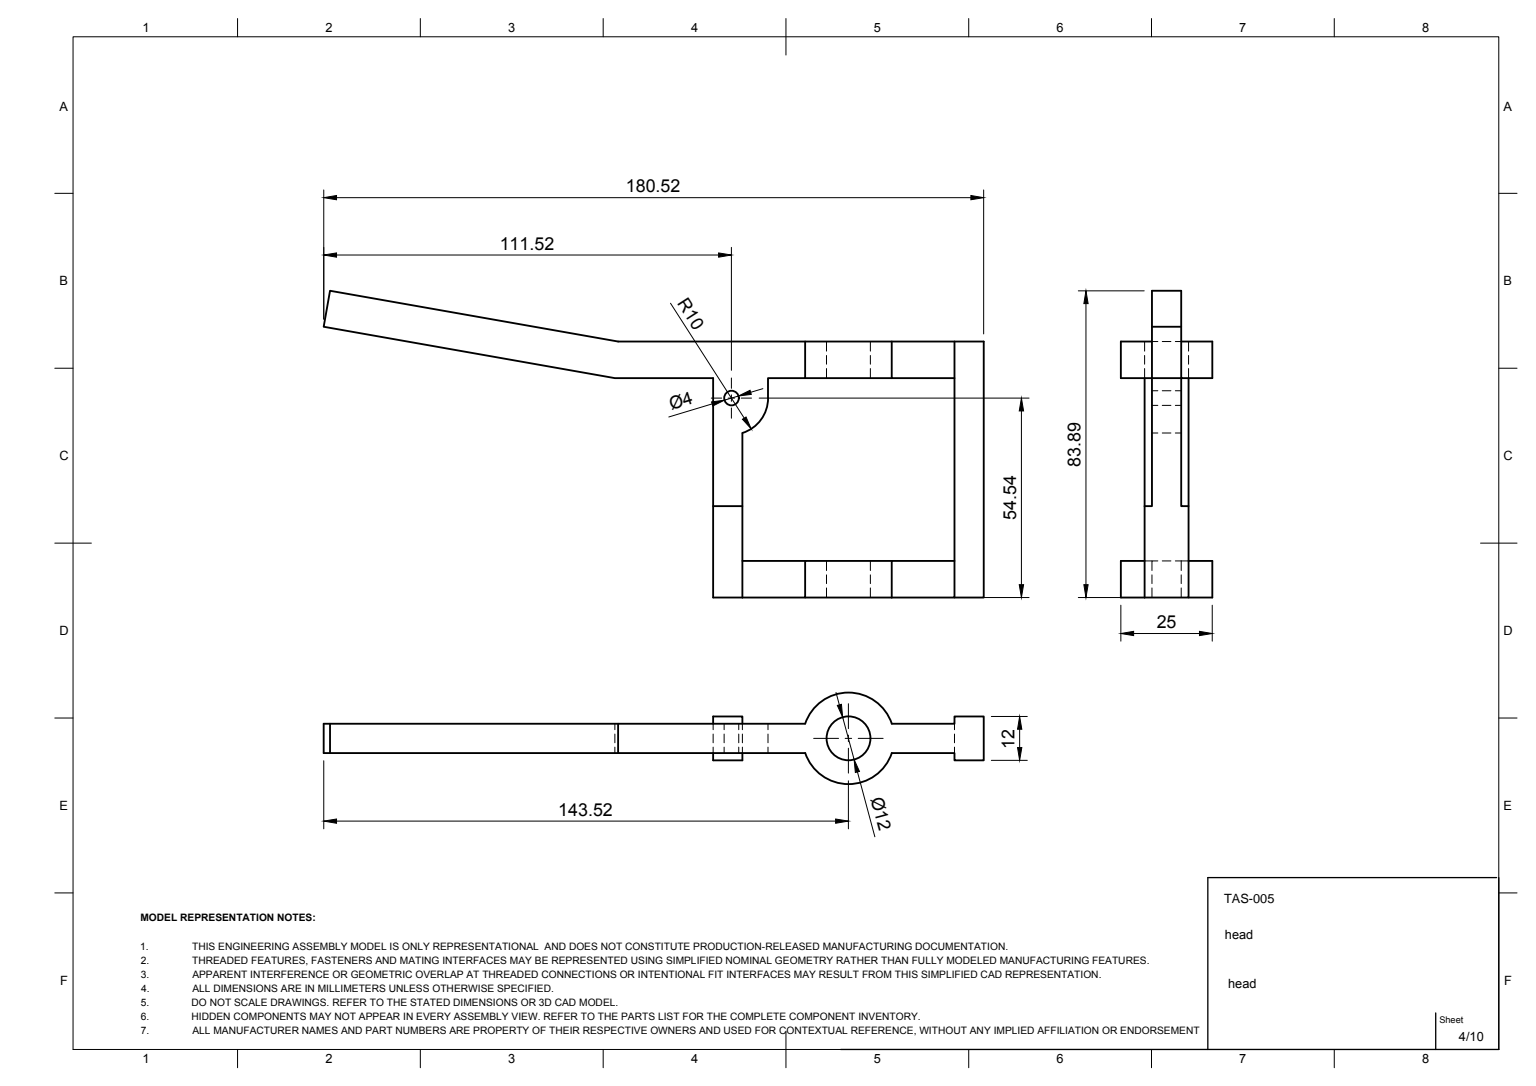
ISO-10303-21;
HEADER;
/* Generated by software containing ST-Developer
 * from STEP Tools, Inc. (www.steptools.com) 
 */

FILE_DESCRIPTION(
/* description */ ('STEP AP214'),
/* implementation_level */ '2;1');

FILE_NAME(
/* name */ 'head.step',
/* time_stamp */ '2026-11-04T19:54:22-08:00',
/* author */ (''),
/* organization */ (''),
/* preprocessor_version */ 'ST-DEVELOPER v20.2',
/* originating_system */ 'Autodesk Translation Framework v15.17.0.0',
/* authorisation */ '');

FILE_SCHEMA (('AUTOMOTIVE_DESIGN { 1 0 10303 214 3 1 1 }'));
ENDSEC;

DATA;
#10=MECHANICAL_DESIGN_GEOMETRIC_PRESENTATION_REPRESENTATION('',(#240),#14084);
#222=SHAPE_REPRESENTATION_RELATIONSHIP('SRR','None',#14121,#231);
#231=ADVANCED_BREP_SHAPE_REPRESENTATION('',(#249),#14076);
#240=STYLED_ITEM('',(#14175),#249);
#249=MANIFOLD_SOLID_BREP('Body1',#3466);
#259=FACE_BOUND('',#580,.T.);
#260=FACE_BOUND('',#590,.T.);
#261=FACE_BOUND('',#593,.T.);
#262=FACE_BOUND('',#599,.T.);
#263=FACE_BOUND('',#601,.T.);
#264=FACE_BOUND('',#603,.T.);
#297=PLANE('',#3613);
#298=PLANE('',#3614);
#299=PLANE('',#3615);
#300=PLANE('',#3617);
#301=PLANE('',#3618);
#302=PLANE('',#3619);
#303=PLANE('',#3620);
#304=PLANE('',#3621);
#305=PLANE('',#3622);
#306=PLANE('',#3623);
#307=PLANE('',#3624);
#308=PLANE('',#3625);
#309=PLANE('',#3627);
#310=PLANE('',#3628);
#311=PLANE('',#3631);
#312=PLANE('',#3632);
#313=PLANE('',#3633);
#314=PLANE('',#3634);
#315=PLANE('',#3636);
#316=PLANE('',#3638);
#317=PLANE('',#3640);
#318=PLANE('',#3641);
#319=PLANE('',#3642);
#320=PLANE('',#3643);
#321=PLANE('',#3645);
#322=PLANE('',#3646);
#323=PLANE('',#3647);
#380=FACE_OUTER_BOUND('',#572,.T.);
#381=FACE_OUTER_BOUND('',#573,.T.);
#382=FACE_OUTER_BOUND('',#574,.T.);
#383=FACE_OUTER_BOUND('',#575,.T.);
#384=FACE_OUTER_BOUND('',#576,.T.);
#385=FACE_OUTER_BOUND('',#577,.T.);
#386=FACE_OUTER_BOUND('',#578,.T.);
#387=FACE_OUTER_BOUND('',#579,.T.);
#388=FACE_OUTER_BOUND('',#581,.T.);
#389=FACE_OUTER_BOUND('',#582,.T.);
#390=FACE_OUTER_BOUND('',#583,.T.);
#391=FACE_OUTER_BOUND('',#584,.T.);
#392=FACE_OUTER_BOUND('',#585,.T.);
#393=FACE_OUTER_BOUND('',#586,.T.);
#394=FACE_OUTER_BOUND('',#587,.T.);
#395=FACE_OUTER_BOUND('',#588,.T.);
#396=FACE_OUTER_BOUND('',#589,.T.);
#397=FACE_OUTER_BOUND('',#591,.T.);
#398=FACE_OUTER_BOUND('',#592,.T.);
#399=FACE_OUTER_BOUND('',#594,.T.);
#400=FACE_OUTER_BOUND('',#595,.T.);
#401=FACE_OUTER_BOUND('',#596,.T.);
#402=FACE_OUTER_BOUND('',#597,.T.);
#403=FACE_OUTER_BOUND('',#598,.T.);
#404=FACE_OUTER_BOUND('',#600,.T.);
#405=FACE_OUTER_BOUND('',#602,.T.);
#406=FACE_OUTER_BOUND('',#604,.T.);
#407=FACE_OUTER_BOUND('',#605,.T.);
#408=FACE_OUTER_BOUND('',#606,.T.);
#409=FACE_OUTER_BOUND('',#607,.T.);
#410=FACE_OUTER_BOUND('',#608,.T.);
#411=FACE_OUTER_BOUND('',#609,.T.);
#412=FACE_OUTER_BOUND('',#610,.T.);
#413=FACE_OUTER_BOUND('',#611,.T.);
#414=FACE_OUTER_BOUND('',#612,.T.);
#572=EDGE_LOOP('',(#2275,#2276,#2277,#2278));
#573=EDGE_LOOP('',(#2279,#2280,#2281,#2282));
#574=EDGE_LOOP('',(#2283,#2284,#2285,#2286));
#575=EDGE_LOOP('',(#2287,#2288,#2289,#2290));
#576=EDGE_LOOP('',(#2291,#2292,#2293,#2294));
#577=EDGE_LOOP('',(#2295,#2296,#2297,#2298,#2299,#2300,#2301,#2302,#2303,
#2304,#2305,#2306));
#578=EDGE_LOOP('',(#2307,#2308,#2309,#2310));
#579=EDGE_LOOP('',(#2311,#2312,#2313,#2314,#2315,#2316,#2317,#2318,#2319,
#2320,#2321,#2322));
#580=EDGE_LOOP('',(#2323));
#581=EDGE_LOOP('',(#2324,#2325,#2326,#2327));
#582=EDGE_LOOP('',(#2328,#2329,#2330,#2331));
#583=EDGE_LOOP('',(#2332,#2333,#2334,#2335,#2336,#2337,#2338,#2339));
#584=EDGE_LOOP('',(#2340,#2341,#2342,#2343,#2344,#2345,#2346,#2347,#2348,
#2349,#2350,#2351));
#585=EDGE_LOOP('',(#2352,#2353,#2354,#2355));
#586=EDGE_LOOP('',(#2356,#2357,#2358,#2359));
#587=EDGE_LOOP('',(#2360,#2361,#2362,#2363));
#588=EDGE_LOOP('',(#2364,#2365,#2366,#2367));
#589=EDGE_LOOP('',(#2368,#2369,#2370,#2371,#2372,#2373,#2374,#2375));
#590=EDGE_LOOP('',(#2376));
#591=EDGE_LOOP('',(#2377,#2378,#2379,#2380));
#592=EDGE_LOOP('',(#2381,#2382,#2383,#2384,#2385,#2386,#2387,#2388,#2389,
#2390,#2391,#2392,#2393,#2394,#2395,#2396));
#593=EDGE_LOOP('',(#2397));
#594=EDGE_LOOP('',(#2398,#2399,#2400,#2401));
#595=EDGE_LOOP('',(#2402,#2403,#2404,#2405));
#596=EDGE_LOOP('',(#2406,#2407,#2408,#2409));
#597=EDGE_LOOP('',(#2410,#2411,#2412,#2413));
#598=EDGE_LOOP('',(#2414,#2415,#2416,#2417,#2418,#2419,#2420,#2421,#2422,
#2423,#2424,#2425));
#599=EDGE_LOOP('',(#2426));
#600=EDGE_LOOP('',(#2427,#2428,#2429,#2430,#2431,#2432,#2433,#2434,#2435,
#2436,#2437,#2438));
#601=EDGE_LOOP('',(#2439));
#602=EDGE_LOOP('',(#2440,#2441,#2442,#2443,#2444,#2445,#2446,#2447));
#603=EDGE_LOOP('',(#2448));
#604=EDGE_LOOP('',(#2449,#2450,#2451,#2452));
#605=EDGE_LOOP('',(#2453,#2454,#2455,#2456));
#606=EDGE_LOOP('',(#2457,#2458,#2459,#2460));
#607=EDGE_LOOP('',(#2461,#2462,#2463,#2464));
#608=EDGE_LOOP('',(#2465,#2466,#2467,#2468));
#609=EDGE_LOOP('',(#2469,#2470,#2471,#2472));
#610=EDGE_LOOP('',(#2473,#2474,#2475,#2476));
#611=EDGE_LOOP('',(#2477,#2478,#2479,#2480));
#612=EDGE_LOOP('',(#2481,#2482,#2483,#2484));
#806=LINE('',#4788,#1063);
#807=LINE('',#4794,#1064);
#808=LINE('',#4800,#1065);
#809=LINE('',#4807,#1066);
#810=LINE('',#4810,#1067);
#811=LINE('',#4816,#1068);
#812=LINE('',#4819,#1069);
#813=LINE('',#4823,#1070);
#814=LINE('',#4825,#1071);
#815=LINE('',#4827,#1072);
#816=LINE('',#4829,#1073);
#817=LINE('',#4831,#1074);
#818=LINE('',#4833,#1075);
#819=LINE('',#4835,#1076);
#820=LINE('',#4837,#1077);
#821=LINE('',#4839,#1078);
#822=LINE('',#4841,#1079);
#823=LINE('',#4843,#1080);
#824=LINE('',#4844,#1081);
#825=LINE('',#4847,#1082);
#826=LINE('',#4849,#1083);
#827=LINE('',#4850,#1084);
#828=LINE('',#4853,#1085);
#829=LINE('',#4855,#1086);
#830=LINE('',#4857,#1087);
#831=LINE('',#4861,#1088);
#832=LINE('',#4863,#1089);
#833=LINE('',#4865,#1090);
#834=LINE('',#4867,#1091);
#835=LINE('',#4869,#1092);
#836=LINE('',#4871,#1093);
#837=LINE('',#4872,#1094);
#838=LINE('',#4875,#1095);
#839=LINE('',#4876,#1096);
#840=LINE('',#4879,#1097);
#841=LINE('',#4881,#1098);
#842=LINE('',#4882,#1099);
#843=LINE('',#4886,#1100);
#844=LINE('',#4888,#1101);
#845=LINE('',#4889,#1102);
#846=LINE('',#4891,#1103);
#847=LINE('',#4893,#1104);
#848=LINE('',#4895,#1105);
#849=LINE('',#4896,#1106);
#850=LINE('',#4899,#1107);
#851=LINE('',#4901,#1108);
#852=LINE('',#4903,#1109);
#853=LINE('',#4905,#1110);
#854=LINE('',#4907,#1111);
#855=LINE('',#4909,#1112);
#856=LINE('',#4910,#1113);
#857=LINE('',#4911,#1114);
#858=LINE('',#4913,#1115);
#859=LINE('',#4914,#1116);
#860=LINE('',#4917,#1117);
#861=LINE('',#4919,#1118);
#862=LINE('',#4920,#1119);
#863=LINE('',#4922,#1120);
#864=LINE('',#4923,#1121);
#865=LINE('',#4926,#1122);
#866=LINE('',#4928,#1123);
#867=LINE('',#4929,#1124);
#868=LINE('',#4934,#1125);
#869=LINE('',#4936,#1126);
#870=LINE('',#4937,#1127);
#871=LINE('',#4939,#1128);
#872=LINE('',#4940,#1129);
#873=LINE('',#4942,#1130);
#874=LINE('',#4945,#1131);
#875=LINE('',#4951,#1132);
#876=LINE('',#4953,#1133);
#877=LINE('',#4955,#1134);
#878=LINE('',#4957,#1135);
#879=LINE('',#4959,#1136);
#880=LINE('',#4960,#1137);
#881=LINE('',#4961,#1138);
#882=LINE('',#4966,#1139);
#883=LINE('',#4968,#1140);
#884=LINE('',#4969,#1141);
#885=LINE('',#4971,#1142);
#886=LINE('',#4973,#1143);
#887=LINE('',#4975,#1144);
#888=LINE('',#4976,#1145);
#889=LINE('',#4977,#1146);
#890=LINE('',#4979,#1147);
#891=LINE('',#4982,#1148);
#892=LINE('',#4984,#1149);
#893=LINE('',#4986,#1150);
#894=LINE('',#4992,#1151);
#1063=VECTOR('',#3949,2.);
#1064=VECTOR('',#3956,6.);
#1065=VECTOR('',#3963,6.);
#1066=VECTOR('',#3970,1000.);
#1067=VECTOR('',#3973,1000.);
#1068=VECTOR('',#3978,1000.);
#1069=VECTOR('',#3981,1000.);
#1070=VECTOR('',#3984,1000.);
#1071=VECTOR('',#3985,1000.);
#1072=VECTOR('',#3986,1000.);
#1073=VECTOR('',#3987,1000.);
#1074=VECTOR('',#3988,1000.);
#1075=VECTOR('',#3989,1000.);
#1076=VECTOR('',#3990,1000.);
#1077=VECTOR('',#3991,1000.);
#1078=VECTOR('',#3992,1000.);
#1079=VECTOR('',#3993,1000.);
#1080=VECTOR('',#3994,1000.);
#1081=VECTOR('',#3995,1000.);
#1082=VECTOR('',#3998,1000.);
#1083=VECTOR('',#3999,1000.);
#1084=VECTOR('',#4000,1000.);
#1085=VECTOR('',#4003,1000.);
#1086=VECTOR('',#4004,1000.);
#1087=VECTOR('',#4005,1000.);
#1088=VECTOR('',#4008,1000.);
#1089=VECTOR('',#4009,1000.);
#1090=VECTOR('',#4010,1000.);
#1091=VECTOR('',#4011,1000.);
#1092=VECTOR('',#4012,1000.);
#1093=VECTOR('',#4013,1000.);
#1094=VECTOR('',#4014,1000.);
#1095=VECTOR('',#4017,1000.);
#1096=VECTOR('',#4018,1000.);
#1097=VECTOR('',#4021,1000.);
#1098=VECTOR('',#4022,1000.);
#1099=VECTOR('',#4023,1000.);
#1100=VECTOR('',#4026,1000.);
#1101=VECTOR('',#4027,1000.);
#1102=VECTOR('',#4028,1000.);
#1103=VECTOR('',#4029,1000.);
#1104=VECTOR('',#4030,1000.);
#1105=VECTOR('',#4031,1000.);
#1106=VECTOR('',#4032,1000.);
#1107=VECTOR('',#4035,1000.);
#1108=VECTOR('',#4036,1000.);
#1109=VECTOR('',#4037,1000.);
#1110=VECTOR('',#4038,1000.);
#1111=VECTOR('',#4039,1000.);
#1112=VECTOR('',#4040,1000.);
#1113=VECTOR('',#4041,1000.);
#1114=VECTOR('',#4042,1000.);
#1115=VECTOR('',#4045,1000.);
#1116=VECTOR('',#4046,1000.);
#1117=VECTOR('',#4049,1000.);
#1118=VECTOR('',#4050,1000.);
#1119=VECTOR('',#4051,1000.);
#1120=VECTOR('',#4054,1000.);
#1121=VECTOR('',#4055,1000.);
#1122=VECTOR('',#4058,1000.);
#1123=VECTOR('',#4059,1000.);
#1124=VECTOR('',#4060,1000.);
#1125=VECTOR('',#4067,1000.);
#1126=VECTOR('',#4068,1000.);
#1127=VECTOR('',#4069,1000.);
#1128=VECTOR('',#4072,1000.);
#1129=VECTOR('',#4073,1000.);
#1130=VECTOR('',#4076,1000.);
#1131=VECTOR('',#4081,1000.);
#1132=VECTOR('',#4088,1000.);
#1133=VECTOR('',#4091,1000.);
#1134=VECTOR('',#4092,1000.);
#1135=VECTOR('',#4093,1000.);
#1136=VECTOR('',#4094,1000.);
#1137=VECTOR('',#4095,1000.);
#1138=VECTOR('',#4096,1000.);
#1139=VECTOR('',#4101,1000.);
#1140=VECTOR('',#4102,1000.);
#1141=VECTOR('',#4103,1000.);
#1142=VECTOR('',#4104,1000.);
#1143=VECTOR('',#4105,1000.);
#1144=VECTOR('',#4106,1000.);
#1145=VECTOR('',#4107,1000.);
#1146=VECTOR('',#4108,1000.);
#1147=VECTOR('',#4111,1000.);
#1148=VECTOR('',#4116,1000.);
#1149=VECTOR('',#4119,1000.);
#1150=VECTOR('',#4122,1000.);
#1151=VECTOR('',#4133,1000.);
#1293=CIRCLE('',#3599,2.);
#1294=CIRCLE('',#3600,2.);
#1295=CIRCLE('',#3602,6.);
#1296=CIRCLE('',#3603,6.);
#1297=CIRCLE('',#3605,6.);
#1298=CIRCLE('',#3606,6.);
#1299=CIRCLE('',#3608,12.5);
#1300=CIRCLE('',#3609,12.5);
#1301=CIRCLE('',#3611,12.5);
#1302=CIRCLE('',#3612,12.5);
#1303=CIRCLE('',#3616,12.5);
#1304=CIRCLE('',#3626,12.5);
#1305=CIRCLE('',#3629,12.5);
#1306=CIRCLE('',#3635,10.);
#1307=CIRCLE('',#3637,10.);
#1308=CIRCLE('',#3639,12.5);
#1403=VERTEX_POINT('',#4785);
#1404=VERTEX_POINT('',#4787);
#1405=VERTEX_POINT('',#4791);
#1406=VERTEX_POINT('',#4793);
#1407=VERTEX_POINT('',#4797);
#1408=VERTEX_POINT('',#4799);
#1409=VERTEX_POINT('',#4803);
#1410=VERTEX_POINT('',#4804);
#1411=VERTEX_POINT('',#4806);
#1412=VERTEX_POINT('',#4808);
#1413=VERTEX_POINT('',#4812);
#1414=VERTEX_POINT('',#4813);
#1415=VERTEX_POINT('',#4815);
#1416=VERTEX_POINT('',#4817);
#1417=VERTEX_POINT('',#4821);
#1418=VERTEX_POINT('',#4822);
#1419=VERTEX_POINT('',#4824);
#1420=VERTEX_POINT('',#4826);
#1421=VERTEX_POINT('',#4828);
#1422=VERTEX_POINT('',#4830);
#1423=VERTEX_POINT('',#4832);
#1424=VERTEX_POINT('',#4834);
#1425=VERTEX_POINT('',#4836);
#1426=VERTEX_POINT('',#4838);
#1427=VERTEX_POINT('',#4840);
#1428=VERTEX_POINT('',#4842);
#1429=VERTEX_POINT('',#4846);
#1430=VERTEX_POINT('',#4848);
#1431=VERTEX_POINT('',#4852);
#1432=VERTEX_POINT('',#4854);
#1433=VERTEX_POINT('',#4856);
#1434=VERTEX_POINT('',#4858);
#1435=VERTEX_POINT('',#4860);
#1436=VERTEX_POINT('',#4862);
#1437=VERTEX_POINT('',#4864);
#1438=VERTEX_POINT('',#4866);
#1439=VERTEX_POINT('',#4868);
#1440=VERTEX_POINT('',#4870);
#1441=VERTEX_POINT('',#4874);
#1442=VERTEX_POINT('',#4878);
#1443=VERTEX_POINT('',#4880);
#1444=VERTEX_POINT('',#4884);
#1445=VERTEX_POINT('',#4885);
#1446=VERTEX_POINT('',#4887);
#1447=VERTEX_POINT('',#4890);
#1448=VERTEX_POINT('',#4892);
#1449=VERTEX_POINT('',#4894);
#1450=VERTEX_POINT('',#4898);
#1451=VERTEX_POINT('',#4900);
#1452=VERTEX_POINT('',#4902);
#1453=VERTEX_POINT('',#4904);
#1454=VERTEX_POINT('',#4906);
#1455=VERTEX_POINT('',#4908);
#1456=VERTEX_POINT('',#4916);
#1457=VERTEX_POINT('',#4918);
#1458=VERTEX_POINT('',#4925);
#1459=VERTEX_POINT('',#4927);
#1460=VERTEX_POINT('',#4933);
#1461=VERTEX_POINT('',#4935);
#1462=VERTEX_POINT('',#4949);
#1463=VERTEX_POINT('',#4950);
#1464=VERTEX_POINT('',#4954);
#1465=VERTEX_POINT('',#4956);
#1466=VERTEX_POINT('',#4958);
#1467=VERTEX_POINT('',#4963);
#1468=VERTEX_POINT('',#4965);
#1469=VERTEX_POINT('',#4967);
#1470=VERTEX_POINT('',#4970);
#1471=VERTEX_POINT('',#4972);
#1472=VERTEX_POINT('',#4974);
#1741=EDGE_CURVE('',#1403,#1403,#1293,.T.);
#1742=EDGE_CURVE('',#1403,#1404,#806,.T.);
#1743=EDGE_CURVE('',#1404,#1404,#1294,.T.);
#1744=EDGE_CURVE('',#1405,#1405,#1295,.T.);
#1745=EDGE_CURVE('',#1405,#1406,#807,.T.);
#1746=EDGE_CURVE('',#1406,#1406,#1296,.T.);
#1747=EDGE_CURVE('',#1407,#1407,#1297,.T.);
#1748=EDGE_CURVE('',#1407,#1408,#808,.T.);
#1749=EDGE_CURVE('',#1408,#1408,#1298,.T.);
#1750=EDGE_CURVE('',#1409,#1410,#1299,.T.);
#1751=EDGE_CURVE('',#1411,#1410,#809,.T.);
#1752=EDGE_CURVE('',#1412,#1411,#1300,.T.);
#1753=EDGE_CURVE('',#1409,#1412,#810,.T.);
#1754=EDGE_CURVE('',#1413,#1414,#1301,.T.);
#1755=EDGE_CURVE('',#1415,#1414,#811,.T.);
#1756=EDGE_CURVE('',#1416,#1415,#1302,.T.);
#1757=EDGE_CURVE('',#1413,#1416,#812,.T.);
#1758=EDGE_CURVE('',#1417,#1418,#813,.T.);
#1759=EDGE_CURVE('',#1418,#1419,#814,.T.);
#1760=EDGE_CURVE('',#1420,#1419,#815,.T.);
#1761=EDGE_CURVE('',#1421,#1420,#816,.T.);
#1762=EDGE_CURVE('',#1421,#1422,#817,.T.);
#1763=EDGE_CURVE('',#1422,#1423,#818,.T.);
#1764=EDGE_CURVE('',#1424,#1423,#819,.T.);
#1765=EDGE_CURVE('',#1424,#1425,#820,.T.);
#1766=EDGE_CURVE('',#1425,#1426,#821,.T.);
#1767=EDGE_CURVE('',#1426,#1427,#822,.T.);
#1768=EDGE_CURVE('',#1428,#1427,#823,.T.);
#1769=EDGE_CURVE('',#1417,#1428,#824,.T.);
#1770=EDGE_CURVE('',#1428,#1429,#825,.T.);
#1771=EDGE_CURVE('',#1427,#1430,#826,.T.);
#1772=EDGE_CURVE('',#1429,#1430,#827,.T.);
#1773=EDGE_CURVE('',#1411,#1431,#828,.T.);
#1774=EDGE_CURVE('',#1431,#1432,#829,.T.);
#1775=EDGE_CURVE('',#1433,#1432,#830,.T.);
#1776=EDGE_CURVE('',#1433,#1434,#1303,.T.);
#1777=EDGE_CURVE('',#1435,#1434,#831,.T.);
#1778=EDGE_CURVE('',#1435,#1436,#832,.T.);
#1779=EDGE_CURVE('',#1436,#1437,#833,.T.);
#1780=EDGE_CURVE('',#1437,#1438,#834,.T.);
#1781=EDGE_CURVE('',#1438,#1439,#835,.T.);
#1782=EDGE_CURVE('',#1439,#1440,#836,.T.);
#1783=EDGE_CURVE('',#1440,#1412,#837,.T.);
#1784=EDGE_CURVE('',#1441,#1409,#838,.T.);
#1785=EDGE_CURVE('',#1440,#1441,#839,.T.);
#1786=EDGE_CURVE('',#1442,#1434,#840,.T.);
#1787=EDGE_CURVE('',#1443,#1442,#841,.T.);
#1788=EDGE_CURVE('',#1435,#1443,#842,.T.);
#1789=EDGE_CURVE('',#1444,#1445,#843,.T.);
#1790=EDGE_CURVE('',#1446,#1445,#844,.T.);
#1791=EDGE_CURVE('',#1429,#1446,#845,.T.);
#1792=EDGE_CURVE('',#1447,#1430,#846,.T.);
#1793=EDGE_CURVE('',#1448,#1447,#847,.T.);
#1794=EDGE_CURVE('',#1449,#1448,#848,.T.);
#1795=EDGE_CURVE('',#1444,#1449,#849,.T.);
#1796=EDGE_CURVE('',#1439,#1450,#850,.T.);
#1797=EDGE_CURVE('',#1450,#1451,#851,.T.);
#1798=EDGE_CURVE('',#1451,#1452,#852,.T.);
#1799=EDGE_CURVE('',#1452,#1453,#853,.T.);
#1800=EDGE_CURVE('',#1454,#1453,#854,.T.);
#1801=EDGE_CURVE('',#1454,#1455,#855,.T.);
#1802=EDGE_CURVE('',#1436,#1455,#856,.T.);
#1803=EDGE_CURVE('',#1441,#1443,#857,.T.);
#1804=EDGE_CURVE('',#1451,#1413,#858,.T.);
#1805=EDGE_CURVE('',#1452,#1416,#859,.T.);
#1806=EDGE_CURVE('',#1454,#1456,#860,.T.);
#1807=EDGE_CURVE('',#1453,#1457,#861,.T.);
#1808=EDGE_CURVE('',#1456,#1457,#862,.T.);
#1809=EDGE_CURVE('',#1415,#1425,#863,.T.);
#1810=EDGE_CURVE('',#1414,#1426,#864,.T.);
#1811=EDGE_CURVE('',#1458,#1424,#865,.T.);
#1812=EDGE_CURVE('',#1459,#1423,#866,.T.);
#1813=EDGE_CURVE('',#1458,#1459,#867,.T.);
#1814=EDGE_CURVE('',#1458,#1457,#1304,.T.);
#1815=EDGE_CURVE('',#1438,#1460,#868,.T.);
#1816=EDGE_CURVE('',#1437,#1461,#869,.T.);
#1817=EDGE_CURVE('',#1460,#1461,#870,.T.);
#1818=EDGE_CURVE('',#1460,#1450,#871,.T.);
#1819=EDGE_CURVE('',#1455,#1461,#872,.T.);
#1820=EDGE_CURVE('',#1459,#1456,#1305,.T.);
#1821=EDGE_CURVE('',#1447,#1422,#873,.T.);
#1822=EDGE_CURVE('',#1421,#1448,#874,.T.);
#1823=EDGE_CURVE('',#1462,#1463,#875,.T.);
#1824=EDGE_CURVE('',#1463,#1418,#1306,.T.);
#1825=EDGE_CURVE('',#1417,#1446,#876,.T.);
#1826=EDGE_CURVE('',#1445,#1464,#877,.T.);
#1827=EDGE_CURVE('',#1464,#1465,#878,.T.);
#1828=EDGE_CURVE('',#1466,#1465,#879,.T.);
#1829=EDGE_CURVE('',#1431,#1466,#880,.T.);
#1830=EDGE_CURVE('',#1410,#1462,#881,.T.);
#1831=EDGE_CURVE('',#1419,#1467,#1307,.T.);
#1832=EDGE_CURVE('',#1468,#1467,#882,.T.);
#1833=EDGE_CURVE('',#1469,#1468,#883,.T.);
#1834=EDGE_CURVE('',#1433,#1469,#884,.T.);
#1835=EDGE_CURVE('',#1432,#1470,#885,.T.);
#1836=EDGE_CURVE('',#1470,#1471,#886,.T.);
#1837=EDGE_CURVE('',#1472,#1471,#887,.T.);
#1838=EDGE_CURVE('',#1444,#1472,#888,.T.);
#1839=EDGE_CURVE('',#1420,#1449,#889,.T.);
#1840=EDGE_CURVE('',#1468,#1462,#890,.T.);
#1841=EDGE_CURVE('',#1469,#1442,#1308,.T.);
#1842=EDGE_CURVE('',#1464,#1472,#891,.T.);
#1843=EDGE_CURVE('',#1465,#1471,#892,.T.);
#1844=EDGE_CURVE('',#1466,#1470,#893,.T.);
#1845=EDGE_CURVE('',#1467,#1463,#894,.T.);
#2275=ORIENTED_EDGE('',*,*,#1741,.T.);
#2276=ORIENTED_EDGE('',*,*,#1742,.T.);
#2277=ORIENTED_EDGE('',*,*,#1743,.F.);
#2278=ORIENTED_EDGE('',*,*,#1742,.F.);
#2279=ORIENTED_EDGE('',*,*,#1744,.F.);
#2280=ORIENTED_EDGE('',*,*,#1745,.T.);
#2281=ORIENTED_EDGE('',*,*,#1746,.F.);
#2282=ORIENTED_EDGE('',*,*,#1745,.F.);
#2283=ORIENTED_EDGE('',*,*,#1747,.F.);
#2284=ORIENTED_EDGE('',*,*,#1748,.T.);
#2285=ORIENTED_EDGE('',*,*,#1749,.T.);
#2286=ORIENTED_EDGE('',*,*,#1748,.F.);
#2287=ORIENTED_EDGE('',*,*,#1750,.T.);
#2288=ORIENTED_EDGE('',*,*,#1751,.F.);
#2289=ORIENTED_EDGE('',*,*,#1752,.F.);
#2290=ORIENTED_EDGE('',*,*,#1753,.F.);
#2291=ORIENTED_EDGE('',*,*,#1754,.T.);
#2292=ORIENTED_EDGE('',*,*,#1755,.F.);
#2293=ORIENTED_EDGE('',*,*,#1756,.F.);
#2294=ORIENTED_EDGE('',*,*,#1757,.F.);
#2295=ORIENTED_EDGE('',*,*,#1758,.T.);
#2296=ORIENTED_EDGE('',*,*,#1759,.T.);
#2297=ORIENTED_EDGE('',*,*,#1760,.F.);
#2298=ORIENTED_EDGE('',*,*,#1761,.F.);
#2299=ORIENTED_EDGE('',*,*,#1762,.T.);
#2300=ORIENTED_EDGE('',*,*,#1763,.T.);
#2301=ORIENTED_EDGE('',*,*,#1764,.F.);
#2302=ORIENTED_EDGE('',*,*,#1765,.T.);
#2303=ORIENTED_EDGE('',*,*,#1766,.T.);
#2304=ORIENTED_EDGE('',*,*,#1767,.T.);
#2305=ORIENTED_EDGE('',*,*,#1768,.F.);
#2306=ORIENTED_EDGE('',*,*,#1769,.F.);
#2307=ORIENTED_EDGE('',*,*,#1770,.F.);
#2308=ORIENTED_EDGE('',*,*,#1768,.T.);
#2309=ORIENTED_EDGE('',*,*,#1771,.T.);
#2310=ORIENTED_EDGE('',*,*,#1772,.F.);
#2311=ORIENTED_EDGE('',*,*,#1752,.T.);
#2312=ORIENTED_EDGE('',*,*,#1773,.T.);
#2313=ORIENTED_EDGE('',*,*,#1774,.T.);
#2314=ORIENTED_EDGE('',*,*,#1775,.F.);
#2315=ORIENTED_EDGE('',*,*,#1776,.T.);
#2316=ORIENTED_EDGE('',*,*,#1777,.F.);
#2317=ORIENTED_EDGE('',*,*,#1778,.T.);
#2318=ORIENTED_EDGE('',*,*,#1779,.T.);
#2319=ORIENTED_EDGE('',*,*,#1780,.T.);
#2320=ORIENTED_EDGE('',*,*,#1781,.T.);
#2321=ORIENTED_EDGE('',*,*,#1782,.T.);
#2322=ORIENTED_EDGE('',*,*,#1783,.T.);
#2323=ORIENTED_EDGE('',*,*,#1749,.F.);
#2324=ORIENTED_EDGE('',*,*,#1784,.T.);
#2325=ORIENTED_EDGE('',*,*,#1753,.T.);
#2326=ORIENTED_EDGE('',*,*,#1783,.F.);
#2327=ORIENTED_EDGE('',*,*,#1785,.T.);
#2328=ORIENTED_EDGE('',*,*,#1786,.F.);
#2329=ORIENTED_EDGE('',*,*,#1787,.F.);
#2330=ORIENTED_EDGE('',*,*,#1788,.F.);
#2331=ORIENTED_EDGE('',*,*,#1777,.T.);
#2332=ORIENTED_EDGE('',*,*,#1789,.T.);
#2333=ORIENTED_EDGE('',*,*,#1790,.F.);
#2334=ORIENTED_EDGE('',*,*,#1791,.F.);
#2335=ORIENTED_EDGE('',*,*,#1772,.T.);
#2336=ORIENTED_EDGE('',*,*,#1792,.F.);
#2337=ORIENTED_EDGE('',*,*,#1793,.F.);
#2338=ORIENTED_EDGE('',*,*,#1794,.F.);
#2339=ORIENTED_EDGE('',*,*,#1795,.F.);
#2340=ORIENTED_EDGE('',*,*,#1785,.F.);
#2341=ORIENTED_EDGE('',*,*,#1782,.F.);
#2342=ORIENTED_EDGE('',*,*,#1796,.T.);
#2343=ORIENTED_EDGE('',*,*,#1797,.T.);
#2344=ORIENTED_EDGE('',*,*,#1798,.T.);
#2345=ORIENTED_EDGE('',*,*,#1799,.T.);
#2346=ORIENTED_EDGE('',*,*,#1800,.F.);
#2347=ORIENTED_EDGE('',*,*,#1801,.T.);
#2348=ORIENTED_EDGE('',*,*,#1802,.F.);
#2349=ORIENTED_EDGE('',*,*,#1778,.F.);
#2350=ORIENTED_EDGE('',*,*,#1788,.T.);
#2351=ORIENTED_EDGE('',*,*,#1803,.F.);
#2352=ORIENTED_EDGE('',*,*,#1798,.F.);
#2353=ORIENTED_EDGE('',*,*,#1804,.T.);
#2354=ORIENTED_EDGE('',*,*,#1757,.T.);
#2355=ORIENTED_EDGE('',*,*,#1805,.F.);
#2356=ORIENTED_EDGE('',*,*,#1806,.F.);
#2357=ORIENTED_EDGE('',*,*,#1800,.T.);
#2358=ORIENTED_EDGE('',*,*,#1807,.T.);
#2359=ORIENTED_EDGE('',*,*,#1808,.F.);
#2360=ORIENTED_EDGE('',*,*,#1766,.F.);
#2361=ORIENTED_EDGE('',*,*,#1809,.F.);
#2362=ORIENTED_EDGE('',*,*,#1755,.T.);
#2363=ORIENTED_EDGE('',*,*,#1810,.T.);
#2364=ORIENTED_EDGE('',*,*,#1811,.T.);
#2365=ORIENTED_EDGE('',*,*,#1764,.T.);
#2366=ORIENTED_EDGE('',*,*,#1812,.F.);
#2367=ORIENTED_EDGE('',*,*,#1813,.F.);
#2368=ORIENTED_EDGE('',*,*,#1799,.F.);
#2369=ORIENTED_EDGE('',*,*,#1805,.T.);
#2370=ORIENTED_EDGE('',*,*,#1756,.T.);
#2371=ORIENTED_EDGE('',*,*,#1809,.T.);
#2372=ORIENTED_EDGE('',*,*,#1765,.F.);
#2373=ORIENTED_EDGE('',*,*,#1811,.F.);
#2374=ORIENTED_EDGE('',*,*,#1814,.T.);
#2375=ORIENTED_EDGE('',*,*,#1807,.F.);
#2376=ORIENTED_EDGE('',*,*,#1746,.T.);
#2377=ORIENTED_EDGE('',*,*,#1815,.F.);
#2378=ORIENTED_EDGE('',*,*,#1780,.F.);
#2379=ORIENTED_EDGE('',*,*,#1816,.T.);
#2380=ORIENTED_EDGE('',*,*,#1817,.F.);
#2381=ORIENTED_EDGE('',*,*,#1792,.T.);
#2382=ORIENTED_EDGE('',*,*,#1771,.F.);
#2383=ORIENTED_EDGE('',*,*,#1767,.F.);
#2384=ORIENTED_EDGE('',*,*,#1810,.F.);
#2385=ORIENTED_EDGE('',*,*,#1754,.F.);
#2386=ORIENTED_EDGE('',*,*,#1804,.F.);
#2387=ORIENTED_EDGE('',*,*,#1797,.F.);
#2388=ORIENTED_EDGE('',*,*,#1818,.F.);
#2389=ORIENTED_EDGE('',*,*,#1817,.T.);
#2390=ORIENTED_EDGE('',*,*,#1819,.F.);
#2391=ORIENTED_EDGE('',*,*,#1801,.F.);
#2392=ORIENTED_EDGE('',*,*,#1806,.T.);
#2393=ORIENTED_EDGE('',*,*,#1820,.F.);
#2394=ORIENTED_EDGE('',*,*,#1812,.T.);
#2395=ORIENTED_EDGE('',*,*,#1763,.F.);
#2396=ORIENTED_EDGE('',*,*,#1821,.F.);
#2397=ORIENTED_EDGE('',*,*,#1744,.T.);
#2398=ORIENTED_EDGE('',*,*,#1820,.T.);
#2399=ORIENTED_EDGE('',*,*,#1808,.T.);
#2400=ORIENTED_EDGE('',*,*,#1814,.F.);
#2401=ORIENTED_EDGE('',*,*,#1813,.T.);
#2402=ORIENTED_EDGE('',*,*,#1762,.F.);
#2403=ORIENTED_EDGE('',*,*,#1822,.T.);
#2404=ORIENTED_EDGE('',*,*,#1793,.T.);
#2405=ORIENTED_EDGE('',*,*,#1821,.T.);
#2406=ORIENTED_EDGE('',*,*,#1818,.T.);
#2407=ORIENTED_EDGE('',*,*,#1796,.F.);
#2408=ORIENTED_EDGE('',*,*,#1781,.F.);
#2409=ORIENTED_EDGE('',*,*,#1815,.T.);
#2410=ORIENTED_EDGE('',*,*,#1819,.T.);
#2411=ORIENTED_EDGE('',*,*,#1816,.F.);
#2412=ORIENTED_EDGE('',*,*,#1779,.F.);
#2413=ORIENTED_EDGE('',*,*,#1802,.T.);
#2414=ORIENTED_EDGE('',*,*,#1823,.T.);
#2415=ORIENTED_EDGE('',*,*,#1824,.T.);
#2416=ORIENTED_EDGE('',*,*,#1758,.F.);
#2417=ORIENTED_EDGE('',*,*,#1825,.T.);
#2418=ORIENTED_EDGE('',*,*,#1790,.T.);
#2419=ORIENTED_EDGE('',*,*,#1826,.T.);
#2420=ORIENTED_EDGE('',*,*,#1827,.T.);
#2421=ORIENTED_EDGE('',*,*,#1828,.F.);
#2422=ORIENTED_EDGE('',*,*,#1829,.F.);
#2423=ORIENTED_EDGE('',*,*,#1773,.F.);
#2424=ORIENTED_EDGE('',*,*,#1751,.T.);
#2425=ORIENTED_EDGE('',*,*,#1830,.T.);
#2426=ORIENTED_EDGE('',*,*,#1743,.T.);
#2427=ORIENTED_EDGE('',*,*,#1760,.T.);
#2428=ORIENTED_EDGE('',*,*,#1831,.T.);
#2429=ORIENTED_EDGE('',*,*,#1832,.F.);
#2430=ORIENTED_EDGE('',*,*,#1833,.F.);
#2431=ORIENTED_EDGE('',*,*,#1834,.F.);
#2432=ORIENTED_EDGE('',*,*,#1775,.T.);
#2433=ORIENTED_EDGE('',*,*,#1835,.T.);
#2434=ORIENTED_EDGE('',*,*,#1836,.T.);
#2435=ORIENTED_EDGE('',*,*,#1837,.F.);
#2436=ORIENTED_EDGE('',*,*,#1838,.F.);
#2437=ORIENTED_EDGE('',*,*,#1795,.T.);
#2438=ORIENTED_EDGE('',*,*,#1839,.F.);
#2439=ORIENTED_EDGE('',*,*,#1741,.F.);
#2440=ORIENTED_EDGE('',*,*,#1833,.T.);
#2441=ORIENTED_EDGE('',*,*,#1840,.T.);
#2442=ORIENTED_EDGE('',*,*,#1830,.F.);
#2443=ORIENTED_EDGE('',*,*,#1750,.F.);
#2444=ORIENTED_EDGE('',*,*,#1784,.F.);
#2445=ORIENTED_EDGE('',*,*,#1803,.T.);
#2446=ORIENTED_EDGE('',*,*,#1787,.T.);
#2447=ORIENTED_EDGE('',*,*,#1841,.F.);
#2448=ORIENTED_EDGE('',*,*,#1747,.T.);
#2449=ORIENTED_EDGE('',*,*,#1789,.F.);
#2450=ORIENTED_EDGE('',*,*,#1838,.T.);
#2451=ORIENTED_EDGE('',*,*,#1842,.F.);
#2452=ORIENTED_EDGE('',*,*,#1826,.F.);
#2453=ORIENTED_EDGE('',*,*,#1837,.T.);
#2454=ORIENTED_EDGE('',*,*,#1843,.F.);
#2455=ORIENTED_EDGE('',*,*,#1827,.F.);
#2456=ORIENTED_EDGE('',*,*,#1842,.T.);
#2457=ORIENTED_EDGE('',*,*,#1836,.F.);
#2458=ORIENTED_EDGE('',*,*,#1844,.F.);
#2459=ORIENTED_EDGE('',*,*,#1828,.T.);
#2460=ORIENTED_EDGE('',*,*,#1843,.T.);
#2461=ORIENTED_EDGE('',*,*,#1835,.F.);
#2462=ORIENTED_EDGE('',*,*,#1774,.F.);
#2463=ORIENTED_EDGE('',*,*,#1829,.T.);
#2464=ORIENTED_EDGE('',*,*,#1844,.T.);
#2465=ORIENTED_EDGE('',*,*,#1841,.T.);
#2466=ORIENTED_EDGE('',*,*,#1786,.T.);
#2467=ORIENTED_EDGE('',*,*,#1776,.F.);
#2468=ORIENTED_EDGE('',*,*,#1834,.T.);
#2469=ORIENTED_EDGE('',*,*,#1761,.T.);
#2470=ORIENTED_EDGE('',*,*,#1839,.T.);
#2471=ORIENTED_EDGE('',*,*,#1794,.T.);
#2472=ORIENTED_EDGE('',*,*,#1822,.F.);
#2473=ORIENTED_EDGE('',*,*,#1769,.T.);
#2474=ORIENTED_EDGE('',*,*,#1770,.T.);
#2475=ORIENTED_EDGE('',*,*,#1791,.T.);
#2476=ORIENTED_EDGE('',*,*,#1825,.F.);
#2477=ORIENTED_EDGE('',*,*,#1832,.T.);
#2478=ORIENTED_EDGE('',*,*,#1845,.T.);
#2479=ORIENTED_EDGE('',*,*,#1823,.F.);
#2480=ORIENTED_EDGE('',*,*,#1840,.F.);
#2481=ORIENTED_EDGE('',*,*,#1831,.F.);
#2482=ORIENTED_EDGE('',*,*,#1759,.F.);
#2483=ORIENTED_EDGE('',*,*,#1824,.F.);
#2484=ORIENTED_EDGE('',*,*,#1845,.F.);
#3190=CYLINDRICAL_SURFACE('',#3598,2.);
#3191=CYLINDRICAL_SURFACE('',#3601,6.);
#3192=CYLINDRICAL_SURFACE('',#3604,6.);
#3193=CYLINDRICAL_SURFACE('',#3607,12.5);
#3194=CYLINDRICAL_SURFACE('',#3610,12.5);
#3195=CYLINDRICAL_SURFACE('',#3630,12.5);
#3196=CYLINDRICAL_SURFACE('',#3644,12.5);
#3197=CYLINDRICAL_SURFACE('',#3648,10.);
#3290=ADVANCED_FACE('',(#380),#3190,.F.);
#3291=ADVANCED_FACE('',(#381),#3191,.F.);
#3292=ADVANCED_FACE('',(#382),#3192,.F.);
#3293=ADVANCED_FACE('',(#383),#3193,.T.);
#3294=ADVANCED_FACE('',(#384),#3194,.T.);
#3295=ADVANCED_FACE('',(#385),#297,.F.);
#3296=ADVANCED_FACE('',(#386),#298,.F.);
#3297=ADVANCED_FACE('',(#387,#259),#299,.T.);
#3298=ADVANCED_FACE('',(#388),#300,.F.);
#3299=ADVANCED_FACE('',(#389),#301,.T.);
#3300=ADVANCED_FACE('',(#390),#302,.T.);
#3301=ADVANCED_FACE('',(#391),#303,.F.);
#3302=ADVANCED_FACE('',(#392),#304,.F.);
#3303=ADVANCED_FACE('',(#393),#305,.T.);
#3304=ADVANCED_FACE('',(#394),#306,.F.);
#3305=ADVANCED_FACE('',(#395),#307,.T.);
#3306=ADVANCED_FACE('',(#396,#260),#308,.F.);
#3307=ADVANCED_FACE('',(#397),#309,.T.);
#3308=ADVANCED_FACE('',(#398,#261),#310,.T.);
#3309=ADVANCED_FACE('',(#399),#3195,.T.);
#3310=ADVANCED_FACE('',(#400),#311,.F.);
#3311=ADVANCED_FACE('',(#401),#312,.F.);
#3312=ADVANCED_FACE('',(#402),#313,.F.);
#3313=ADVANCED_FACE('',(#403,#262),#314,.F.);
#3314=ADVANCED_FACE('',(#404,#263),#315,.T.);
#3315=ADVANCED_FACE('',(#405,#264),#316,.F.);
#3316=ADVANCED_FACE('',(#406),#317,.F.);
#3317=ADVANCED_FACE('',(#407),#318,.F.);
#3318=ADVANCED_FACE('',(#408),#319,.T.);
#3319=ADVANCED_FACE('',(#409),#320,.T.);
#3320=ADVANCED_FACE('',(#410),#3196,.T.);
#3321=ADVANCED_FACE('',(#411),#321,.F.);
#3322=ADVANCED_FACE('',(#412),#322,.F.);
#3323=ADVANCED_FACE('',(#413),#323,.T.);
#3324=ADVANCED_FACE('',(#414),#3197,.T.);
#3466=CLOSED_SHELL('',(#3290,#3291,#3292,#3293,#3294,#3295,#3296,#3297,
#3298,#3299,#3300,#3301,#3302,#3303,#3304,#3305,#3306,#3307,#3308,#3309,
#3310,#3311,#3312,#3313,#3314,#3315,#3316,#3317,#3318,#3319,#3320,#3321,
#3322,#3323,#3324));
#3597=AXIS2_PLACEMENT_3D('',#4783,#3943,#3944);
#3598=AXIS2_PLACEMENT_3D('',#4784,#3945,#3946);
#3599=AXIS2_PLACEMENT_3D('',#4786,#3947,#3948);
#3600=AXIS2_PLACEMENT_3D('',#4789,#3950,#3951);
#3601=AXIS2_PLACEMENT_3D('',#4790,#3952,#3953);
#3602=AXIS2_PLACEMENT_3D('',#4792,#3954,#3955);
#3603=AXIS2_PLACEMENT_3D('',#4795,#3957,#3958);
#3604=AXIS2_PLACEMENT_3D('',#4796,#3959,#3960);
#3605=AXIS2_PLACEMENT_3D('',#4798,#3961,#3962);
#3606=AXIS2_PLACEMENT_3D('',#4801,#3964,#3965);
#3607=AXIS2_PLACEMENT_3D('',#4802,#3966,#3967);
#3608=AXIS2_PLACEMENT_3D('',#4805,#3968,#3969);
#3609=AXIS2_PLACEMENT_3D('',#4809,#3971,#3972);
#3610=AXIS2_PLACEMENT_3D('',#4811,#3974,#3975);
#3611=AXIS2_PLACEMENT_3D('',#4814,#3976,#3977);
#3612=AXIS2_PLACEMENT_3D('',#4818,#3979,#3980);
#3613=AXIS2_PLACEMENT_3D('',#4820,#3982,#3983);
#3614=AXIS2_PLACEMENT_3D('',#4845,#3996,#3997);
#3615=AXIS2_PLACEMENT_3D('',#4851,#4001,#4002);
#3616=AXIS2_PLACEMENT_3D('',#4859,#4006,#4007);
#3617=AXIS2_PLACEMENT_3D('',#4873,#4015,#4016);
#3618=AXIS2_PLACEMENT_3D('',#4877,#4019,#4020);
#3619=AXIS2_PLACEMENT_3D('',#4883,#4024,#4025);
#3620=AXIS2_PLACEMENT_3D('',#4897,#4033,#4034);
#3621=AXIS2_PLACEMENT_3D('',#4912,#4043,#4044);
#3622=AXIS2_PLACEMENT_3D('',#4915,#4047,#4048);
#3623=AXIS2_PLACEMENT_3D('',#4921,#4052,#4053);
#3624=AXIS2_PLACEMENT_3D('',#4924,#4056,#4057);
#3625=AXIS2_PLACEMENT_3D('',#4930,#4061,#4062);
#3626=AXIS2_PLACEMENT_3D('',#4931,#4063,#4064);
#3627=AXIS2_PLACEMENT_3D('',#4932,#4065,#4066);
#3628=AXIS2_PLACEMENT_3D('',#4938,#4070,#4071);
#3629=AXIS2_PLACEMENT_3D('',#4941,#4074,#4075);
#3630=AXIS2_PLACEMENT_3D('',#4943,#4077,#4078);
#3631=AXIS2_PLACEMENT_3D('',#4944,#4079,#4080);
#3632=AXIS2_PLACEMENT_3D('',#4946,#4082,#4083);
#3633=AXIS2_PLACEMENT_3D('',#4947,#4084,#4085);
#3634=AXIS2_PLACEMENT_3D('',#4948,#4086,#4087);
#3635=AXIS2_PLACEMENT_3D('',#4952,#4089,#4090);
#3636=AXIS2_PLACEMENT_3D('',#4962,#4097,#4098);
#3637=AXIS2_PLACEMENT_3D('',#4964,#4099,#4100);
#3638=AXIS2_PLACEMENT_3D('',#4978,#4109,#4110);
#3639=AXIS2_PLACEMENT_3D('',#4980,#4112,#4113);
#3640=AXIS2_PLACEMENT_3D('',#4981,#4114,#4115);
#3641=AXIS2_PLACEMENT_3D('',#4983,#4117,#4118);
#3642=AXIS2_PLACEMENT_3D('',#4985,#4120,#4121);
#3643=AXIS2_PLACEMENT_3D('',#4987,#4123,#4124);
#3644=AXIS2_PLACEMENT_3D('',#4988,#4125,#4126);
#3645=AXIS2_PLACEMENT_3D('',#4989,#4127,#4128);
#3646=AXIS2_PLACEMENT_3D('',#4990,#4129,#4130);
#3647=AXIS2_PLACEMENT_3D('',#4991,#4131,#4132);
#3648=AXIS2_PLACEMENT_3D('',#4993,#4134,#4135);
#3943=DIRECTION('axis',(0.,0.,1.));
#3944=DIRECTION('refdir',(1.,0.,0.));
#3945=DIRECTION('center_axis',(0.,0.,1.));
#3946=DIRECTION('ref_axis',(1.,0.,0.));
#3947=DIRECTION('center_axis',(0.,0.,-1.));
#3948=DIRECTION('ref_axis',(-1.,0.,0.));
#3949=DIRECTION('',(0.,0.,1.));
#3950=DIRECTION('center_axis',(0.,0.,-1.));
#3951=DIRECTION('ref_axis',(-1.,0.,0.));
#3952=DIRECTION('center_axis',(0.,1.,0.));
#3953=DIRECTION('ref_axis',(0.,0.,1.));
#3954=DIRECTION('center_axis',(0.,1.,0.));
#3955=DIRECTION('ref_axis',(0.,0.,1.));
#3956=DIRECTION('',(0.,1.,0.));
#3957=DIRECTION('center_axis',(0.,-1.,0.));
#3958=DIRECTION('ref_axis',(0.,0.,-1.));
#3959=DIRECTION('center_axis',(0.,1.,0.));
#3960=DIRECTION('ref_axis',(0.,0.,1.));
#3961=DIRECTION('center_axis',(0.,1.,0.));
#3962=DIRECTION('ref_axis',(0.,0.,1.));
#3963=DIRECTION('',(0.,1.,0.));
#3964=DIRECTION('center_axis',(0.,1.,0.));
#3965=DIRECTION('ref_axis',(0.,0.,1.));
#3966=DIRECTION('center_axis',(0.,1.,0.));
#3967=DIRECTION('ref_axis',(0.,0.,1.));
#3968=DIRECTION('center_axis',(0.,1.,0.));
#3969=DIRECTION('ref_axis',(0.,0.,1.));
#3970=DIRECTION('',(0.,-1.,0.));
#3971=DIRECTION('center_axis',(0.,1.,0.));
#3972=DIRECTION('ref_axis',(0.,0.,1.));
#3973=DIRECTION('',(0.,1.,0.));
#3974=DIRECTION('center_axis',(0.,1.,0.));
#3975=DIRECTION('ref_axis',(0.,0.,1.));
#3976=DIRECTION('center_axis',(0.,1.,0.));
#3977=DIRECTION('ref_axis',(0.,0.,1.));
#3978=DIRECTION('',(0.,-1.,0.));
#3979=DIRECTION('center_axis',(0.,1.,0.));
#3980=DIRECTION('ref_axis',(0.,0.,1.));
#3981=DIRECTION('',(0.,1.,0.));
#3982=DIRECTION('center_axis',(1.,0.,0.));
#3983=DIRECTION('ref_axis',(0.,0.,-1.));
#3984=DIRECTION('',(0.,1.,0.));
#3985=DIRECTION('',(0.,0.,-1.));
#3986=DIRECTION('',(0.,1.,0.));
#3987=DIRECTION('',(0.,0.,1.));
#3988=DIRECTION('',(0.,-1.,0.));
#3989=DIRECTION('',(0.,0.,1.));
#3990=DIRECTION('',(0.,-1.,0.));
#3991=DIRECTION('',(0.,0.,1.));
#3992=DIRECTION('',(0.,-1.,0.));
#3993=DIRECTION('',(0.,0.,1.));
#3994=DIRECTION('',(0.,-1.,0.));
#3995=DIRECTION('',(0.,0.,1.));
#3996=DIRECTION('center_axis',(-2.16840434497101E-16,0.,-1.));
#3997=DIRECTION('ref_axis',(-1.,0.,2.16840434497101E-16));
#3998=DIRECTION('',(1.,0.,0.));
#3999=DIRECTION('',(1.,0.,-2.16840434497101E-16));
#4000=DIRECTION('',(0.,-1.,0.));
#4001=DIRECTION('center_axis',(0.,1.,0.));
#4002=DIRECTION('ref_axis',(0.,0.,1.));
#4003=DIRECTION('',(1.,0.,0.));
#4004=DIRECTION('',(0.,0.,-1.));
#4005=DIRECTION('',(1.,0.,0.));
#4006=DIRECTION('center_axis',(0.,1.,0.));
#4007=DIRECTION('ref_axis',(0.,0.,1.));
#4008=DIRECTION('',(1.,0.,0.));
#4009=DIRECTION('',(0.,0.,-1.));
#4010=DIRECTION('',(-1.,0.,0.));
#4011=DIRECTION('',(0.,0.,1.));
#4012=DIRECTION('',(1.,0.,0.));
#4013=DIRECTION('',(0.,0.,-1.));
#4014=DIRECTION('',(1.,0.,0.));
#4015=DIRECTION('center_axis',(0.,0.,-1.));
#4016=DIRECTION('ref_axis',(-1.,0.,0.));
#4017=DIRECTION('',(1.,0.,0.));
#4018=DIRECTION('',(0.,-1.,0.));
#4019=DIRECTION('center_axis',(0.,0.,-1.));
#4020=DIRECTION('ref_axis',(-1.,0.,0.));
#4021=DIRECTION('',(0.,1.,0.));
#4022=DIRECTION('',(1.,0.,0.));
#4023=DIRECTION('',(0.,-1.,0.));
#4024=DIRECTION('center_axis',(1.,0.,0.));
#4025=DIRECTION('ref_axis',(0.,0.,-1.));
#4026=DIRECTION('',(0.,0.,1.));
#4027=DIRECTION('',(0.,1.,0.));
#4028=DIRECTION('',(0.,0.,-1.));
#4029=DIRECTION('',(0.,0.,1.));
#4030=DIRECTION('',(0.,-1.,0.));
#4031=DIRECTION('',(0.,0.,-1.));
#4032=DIRECTION('',(0.,-1.,0.));
#4033=DIRECTION('center_axis',(-1.,0.,0.));
#4034=DIRECTION('ref_axis',(0.,0.,1.));
#4035=DIRECTION('',(0.,-1.,0.));
#4036=DIRECTION('',(0.,0.,-1.));
#4037=DIRECTION('',(0.,1.,0.));
#4038=DIRECTION('',(0.,0.,-1.));
#4039=DIRECTION('',(0.,1.,0.));
#4040=DIRECTION('',(0.,0.,-1.));
#4041=DIRECTION('',(0.,-1.,0.));
#4042=DIRECTION('',(0.,0.,-1.));
#4043=DIRECTION('center_axis',(0.,0.,-1.));
#4044=DIRECTION('ref_axis',(-1.,0.,0.));
#4045=DIRECTION('',(1.,0.,0.));
#4046=DIRECTION('',(1.,0.,0.));
#4047=DIRECTION('center_axis',(0.,0.,-1.));
#4048=DIRECTION('ref_axis',(-1.,0.,0.));
#4049=DIRECTION('',(1.,0.,0.));
#4050=DIRECTION('',(1.,0.,0.));
#4051=DIRECTION('',(0.,1.,0.));
#4052=DIRECTION('center_axis',(0.,0.,-1.));
#4053=DIRECTION('ref_axis',(-1.,0.,0.));
#4054=DIRECTION('',(1.,0.,0.));
#4055=DIRECTION('',(1.,0.,0.));
#4056=DIRECTION('center_axis',(0.,0.,-1.));
#4057=DIRECTION('ref_axis',(-1.,0.,0.));
#4058=DIRECTION('',(1.,0.,0.));
#4059=DIRECTION('',(1.,0.,0.));
#4060=DIRECTION('',(0.,-1.,0.));
#4061=DIRECTION('center_axis',(0.,-1.,0.));
#4062=DIRECTION('ref_axis',(-1.,0.,0.));
#4063=DIRECTION('center_axis',(0.,1.,0.));
#4064=DIRECTION('ref_axis',(0.,0.,1.));
#4065=DIRECTION('center_axis',(-1.,0.,0.));
#4066=DIRECTION('ref_axis',(0.,0.,1.));
#4067=DIRECTION('',(0.,-1.,0.));
#4068=DIRECTION('',(0.,-1.,0.));
#4069=DIRECTION('',(0.,0.,-1.));
#4070=DIRECTION('center_axis',(0.,-1.,0.));
#4071=DIRECTION('ref_axis',(-1.,0.,0.));
#4072=DIRECTION('',(1.,0.,0.));
#4073=DIRECTION('',(-1.,0.,0.));
#4074=DIRECTION('center_axis',(0.,1.,0.));
#4075=DIRECTION('ref_axis',(0.,0.,1.));
#4076=DIRECTION('',(-1.,0.,2.16840434497101E-16));
#4077=DIRECTION('center_axis',(0.,1.,0.));
#4078=DIRECTION('ref_axis',(1.22464679914735E-16,0.,-1.));
#4079=DIRECTION('center_axis',(2.16840434497101E-16,0.,1.));
#4080=DIRECTION('ref_axis',(1.,0.,-2.16840434497101E-16));
#4081=DIRECTION('',(1.,0.,0.));
#4082=DIRECTION('center_axis',(0.,0.,-1.));
#4083=DIRECTION('ref_axis',(-1.,0.,0.));
#4084=DIRECTION('center_axis',(0.,0.,1.));
#4085=DIRECTION('ref_axis',(1.,0.,0.));
#4086=DIRECTION('center_axis',(0.,0.,-1.));
#4087=DIRECTION('ref_axis',(-1.,0.,0.));
#4088=DIRECTION('',(0.,-1.,0.));
#4089=DIRECTION('center_axis',(0.,0.,1.));
#4090=DIRECTION('ref_axis',(-1.,0.,0.));
#4091=DIRECTION('',(1.,0.,0.));
#4092=DIRECTION('',(1.,0.,0.));
#4093=DIRECTION('',(0.984807753012208,0.173648177666931,0.));
#4094=DIRECTION('',(0.173648177666933,-0.984807753012208,0.));
#4095=DIRECTION('',(0.984807753012208,0.173648177666931,0.));
#4096=DIRECTION('',(1.,0.,0.));
#4097=DIRECTION('center_axis',(0.,0.,-1.));
#4098=DIRECTION('ref_axis',(-1.,0.,0.));
#4099=DIRECTION('center_axis',(0.,0.,-1.));
#4100=DIRECTION('ref_axis',(-1.,0.,0.));
#4101=DIRECTION('',(0.,-1.,0.));
#4102=DIRECTION('',(1.,0.,0.));
#4103=DIRECTION('',(0.,-1.,0.));
#4104=DIRECTION('',(0.984807753012208,0.173648177666931,0.));
#4105=DIRECTION('',(0.173648177666933,-0.984807753012208,0.));
#4106=DIRECTION('',(0.984807753012208,0.173648177666931,0.));
#4107=DIRECTION('',(1.,0.,0.));
#4108=DIRECTION('',(1.,0.,0.));
#4109=DIRECTION('center_axis',(0.,1.,0.));
#4110=DIRECTION('ref_axis',(0.,0.,1.));
#4111=DIRECTION('',(0.,0.,1.));
#4112=DIRECTION('center_axis',(0.,1.,0.));
#4113=DIRECTION('ref_axis',(0.,0.,1.));
#4114=DIRECTION('center_axis',(0.,1.,0.));
#4115=DIRECTION('ref_axis',(0.,0.,1.));
#4116=DIRECTION('',(0.,0.,-1.));
#4117=DIRECTION('center_axis',(-0.173648177666931,0.984807753012208,0.));
#4118=DIRECTION('ref_axis',(-0.984807753012208,-0.173648177666931,0.));
#4119=DIRECTION('',(0.,0.,-1.));
#4120=DIRECTION('center_axis',(0.984807753012208,0.173648177666933,0.));
#4121=DIRECTION('ref_axis',(-0.173648177666933,0.984807753012208,0.));
#4122=DIRECTION('',(0.,0.,-1.));
#4123=DIRECTION('center_axis',(-0.173648177666931,0.984807753012208,0.));
#4124=DIRECTION('ref_axis',(-0.984807753012208,-0.173648177666931,0.));
#4125=DIRECTION('center_axis',(0.,1.,0.));
#4126=DIRECTION('ref_axis',(1.22464679914735E-16,0.,-1.));
#4127=DIRECTION('center_axis',(0.,-1.,0.));
#4128=DIRECTION('ref_axis',(0.,0.,-1.));
#4129=DIRECTION('center_axis',(0.,-1.,0.));
#4130=DIRECTION('ref_axis',(0.,0.,-1.));
#4131=DIRECTION('center_axis',(-1.,0.,0.));
#4132=DIRECTION('ref_axis',(0.,0.,1.));
#4133=DIRECTION('',(0.,0.,1.));
#4134=DIRECTION('center_axis',(0.,0.,1.));
#4135=DIRECTION('ref_axis',(1.,0.,0.));
#4783=CARTESIAN_POINT('',(0.,0.,0.));
#4784=CARTESIAN_POINT('Origin',(32.,329.539392014169,6.2));
#4785=CARTESIAN_POINT('',(30.,329.539392014169,-4.));
#4786=CARTESIAN_POINT('Origin',(32.,329.539392014169,-4.));
#4787=CARTESIAN_POINT('',(30.,329.539392014169,4.));
#4788=CARTESIAN_POINT('',(30.,329.539392014169,6.2));
#4789=CARTESIAN_POINT('Origin',(32.,329.539392014169,4.));
#4790=CARTESIAN_POINT('Origin',(0.,275.,0.));
#4791=CARTESIAN_POINT('',(-7.34788079488412E-16,275.,-6.));
#4792=CARTESIAN_POINT('Origin',(0.,275.,0.));
#4793=CARTESIAN_POINT('',(-7.34788079488412E-16,285.,-6.));
#4794=CARTESIAN_POINT('',(-7.34788079488412E-16,275.,-6.));
#4795=CARTESIAN_POINT('Origin',(0.,285.,0.));
#4796=CARTESIAN_POINT('Origin',(0.,275.,0.));
#4797=CARTESIAN_POINT('',(-7.34788079488412E-16,335.,-6.));
#4798=CARTESIAN_POINT('Origin',(0.,335.,0.));
#4799=CARTESIAN_POINT('',(-7.34788079488412E-16,345.,-6.));
#4800=CARTESIAN_POINT('',(-7.34788079488412E-16,275.,-6.));
#4801=CARTESIAN_POINT('Origin',(0.,345.,0.));
#4802=CARTESIAN_POINT('Origin',(0.,335.,0.));
#4803=CARTESIAN_POINT('',(-11.842719282327,335.,4.));
#4804=CARTESIAN_POINT('',(11.842719282327,335.,4.));
#4805=CARTESIAN_POINT('Origin',(0.,335.,0.));
#4806=CARTESIAN_POINT('',(11.842719282327,345.,4.));
#4807=CARTESIAN_POINT('',(11.842719282327,335.,4.));
#4808=CARTESIAN_POINT('',(-11.842719282327,345.,4.));
#4809=CARTESIAN_POINT('Origin',(0.,345.,0.));
#4810=CARTESIAN_POINT('',(-11.842719282327,335.,4.));
#4811=CARTESIAN_POINT('Origin',(0.,275.,0.));
#4812=CARTESIAN_POINT('',(-11.842719282327,275.,4.));
#4813=CARTESIAN_POINT('',(11.842719282327,275.,4.));
#4814=CARTESIAN_POINT('Origin',(0.,275.,0.));
#4815=CARTESIAN_POINT('',(11.842719282327,285.,4.));
#4816=CARTESIAN_POINT('',(11.842719282327,275.,4.));
#4817=CARTESIAN_POINT('',(-11.842719282327,285.,4.));
#4818=CARTESIAN_POINT('Origin',(0.,285.,0.));
#4819=CARTESIAN_POINT('',(-11.842719282327,275.,4.));
#4820=CARTESIAN_POINT('Origin',(29.,345.,-5.99999999999999));
#4821=CARTESIAN_POINT('',(29.,300.,4.));
#4822=CARTESIAN_POINT('',(29.,320.,4.));
#4823=CARTESIAN_POINT('',(29.,345.,4.));
#4824=CARTESIAN_POINT('',(29.,320.,-4.));
#4825=CARTESIAN_POINT('',(29.,320.,-5.99999999999999));
#4826=CARTESIAN_POINT('',(29.,300.,-4.));
#4827=CARTESIAN_POINT('',(29.,345.,-4.));
#4828=CARTESIAN_POINT('',(29.,300.,-6.));
#4829=CARTESIAN_POINT('',(29.,300.,-4.));
#4830=CARTESIAN_POINT('',(29.,275.,-5.99999999999999));
#4831=CARTESIAN_POINT('',(29.,345.,-5.99999999999999));
#4832=CARTESIAN_POINT('',(29.,275.,-4.));
#4833=CARTESIAN_POINT('',(29.,275.,-5.99999999999999));
#4834=CARTESIAN_POINT('',(29.,285.,-4.));
#4835=CARTESIAN_POINT('',(29.,285.,-4.));
#4836=CARTESIAN_POINT('',(29.,285.,4.));
#4837=CARTESIAN_POINT('',(29.,285.,0.));
#4838=CARTESIAN_POINT('',(29.,275.,4.));
#4839=CARTESIAN_POINT('',(29.,285.,4.));
#4840=CARTESIAN_POINT('',(29.,275.,6.00000000000001));
#4841=CARTESIAN_POINT('',(29.,275.,-5.99999999999999));
#4842=CARTESIAN_POINT('',(29.,300.,6.));
#4843=CARTESIAN_POINT('',(29.,345.,6.00000000000001));
#4844=CARTESIAN_POINT('',(29.,300.,4.));
#4845=CARTESIAN_POINT('Origin',(37.,345.,6.));
#4846=CARTESIAN_POINT('',(37.,300.,6.));
#4847=CARTESIAN_POINT('',(-37.001,300.,6.));
#4848=CARTESIAN_POINT('',(37.,275.,6.));
#4849=CARTESIAN_POINT('',(37.,275.,6.));
#4850=CARTESIAN_POINT('',(37.,345.,6.));
#4851=CARTESIAN_POINT('Origin',(0.,345.,0.));
#4852=CARTESIAN_POINT('',(63.,345.,4.));
#4853=CARTESIAN_POINT('',(-37.,345.,4.));
#4854=CARTESIAN_POINT('',(63.,345.,-4.));
#4855=CARTESIAN_POINT('',(63.,345.,4.));
#4856=CARTESIAN_POINT('',(11.842719282327,345.,-4.));
#4857=CARTESIAN_POINT('',(-37.,345.,-4.));
#4858=CARTESIAN_POINT('',(-11.842719282327,345.,-4.));
#4859=CARTESIAN_POINT('Origin',(0.,345.,0.));
#4860=CARTESIAN_POINT('',(-29.,345.,-4.));
#4861=CARTESIAN_POINT('',(-37.,345.,-4.));
#4862=CARTESIAN_POINT('',(-29.,345.,-5.99999999999999));
#4863=CARTESIAN_POINT('',(-29.,345.,-5.99999999999999));
#4864=CARTESIAN_POINT('',(-37.,345.,-5.99999999999999));
#4865=CARTESIAN_POINT('',(-37.,345.,-5.99999999999999));
#4866=CARTESIAN_POINT('',(-37.,345.,6.00000000000001));
#4867=CARTESIAN_POINT('',(-37.,345.,-5.99999999999999));
#4868=CARTESIAN_POINT('',(-29.,345.,6.00000000000001));
#4869=CARTESIAN_POINT('',(-37.,345.,6.00000000000001));
#4870=CARTESIAN_POINT('',(-29.,345.,4.));
#4871=CARTESIAN_POINT('',(-29.,345.,-5.99999999999999));
#4872=CARTESIAN_POINT('',(-37.,345.,4.));
#4873=CARTESIAN_POINT('Origin',(0.,0.,4.));
#4874=CARTESIAN_POINT('',(-29.,335.,4.));
#4875=CARTESIAN_POINT('',(-37.,335.,4.));
#4876=CARTESIAN_POINT('',(-29.,345.,4.));
#4877=CARTESIAN_POINT('Origin',(0.,0.,-4.));
#4878=CARTESIAN_POINT('',(-11.842719282327,335.,-4.));
#4879=CARTESIAN_POINT('',(-11.842719282327,335.,-4.));
#4880=CARTESIAN_POINT('',(-29.,335.,-4.));
#4881=CARTESIAN_POINT('',(-37.,335.,-4.));
#4882=CARTESIAN_POINT('',(-29.,345.,-4.));
#4883=CARTESIAN_POINT('Origin',(37.,285.,-4.));
#4884=CARTESIAN_POINT('',(37.,335.,-4.));
#4885=CARTESIAN_POINT('',(37.,335.,4.));
#4886=CARTESIAN_POINT('',(37.,335.,-4.));
#4887=CARTESIAN_POINT('',(37.,300.,4.));
#4888=CARTESIAN_POINT('',(37.,345.,4.));
#4889=CARTESIAN_POINT('',(37.,300.,4.));
#4890=CARTESIAN_POINT('',(37.,275.,-6.));
#4891=CARTESIAN_POINT('',(37.,275.,-4.));
#4892=CARTESIAN_POINT('',(37.,300.,-6.));
#4893=CARTESIAN_POINT('',(37.,345.,-6.));
#4894=CARTESIAN_POINT('',(37.,300.,-4.));
#4895=CARTESIAN_POINT('',(37.,300.,-4.));
#4896=CARTESIAN_POINT('',(37.,345.,-4.));
#4897=CARTESIAN_POINT('Origin',(-29.,345.,-5.99999999999999));
#4898=CARTESIAN_POINT('',(-29.,275.,6.00000000000001));
#4899=CARTESIAN_POINT('',(-29.,345.,6.00000000000001));
#4900=CARTESIAN_POINT('',(-29.,275.,4.));
#4901=CARTESIAN_POINT('',(-29.,275.,-5.99999999999999));
#4902=CARTESIAN_POINT('',(-29.,285.,4.));
#4903=CARTESIAN_POINT('',(-29.,285.,4.));
#4904=CARTESIAN_POINT('',(-29.,285.,-4.));
#4905=CARTESIAN_POINT('',(-29.,285.,0.));
#4906=CARTESIAN_POINT('',(-29.,275.,-4.));
#4907=CARTESIAN_POINT('',(-29.,285.,-4.));
#4908=CARTESIAN_POINT('',(-29.,275.,-5.99999999999999));
#4909=CARTESIAN_POINT('',(-29.,275.,-5.99999999999999));
#4910=CARTESIAN_POINT('',(-29.,345.,-5.99999999999999));
#4911=CARTESIAN_POINT('',(-29.,335.,-5.99999999999999));
#4912=CARTESIAN_POINT('Origin',(-37.,285.,4.));
#4913=CARTESIAN_POINT('',(-37.,275.,4.));
#4914=CARTESIAN_POINT('',(-37.,285.,4.));
#4915=CARTESIAN_POINT('Origin',(-37.,285.,-4.));
#4916=CARTESIAN_POINT('',(-11.842719282327,275.,-4.));
#4917=CARTESIAN_POINT('',(-37.,275.,-4.));
#4918=CARTESIAN_POINT('',(-11.842719282327,285.,-4.));
#4919=CARTESIAN_POINT('',(-37.,285.,-4.));
#4920=CARTESIAN_POINT('',(-11.842719282327,275.,-4.));
#4921=CARTESIAN_POINT('Origin',(-37.,285.,4.));
#4922=CARTESIAN_POINT('',(-37.,285.,4.));
#4923=CARTESIAN_POINT('',(-37.,275.,4.));
#4924=CARTESIAN_POINT('Origin',(-37.,285.,-4.));
#4925=CARTESIAN_POINT('',(11.842719282327,285.,-4.));
#4926=CARTESIAN_POINT('',(-37.,285.,-4.));
#4927=CARTESIAN_POINT('',(11.842719282327,275.,-4.));
#4928=CARTESIAN_POINT('',(-37.,275.,-4.));
#4929=CARTESIAN_POINT('',(11.842719282327,275.,-4.));
#4930=CARTESIAN_POINT('Origin',(0.,285.,0.));
#4931=CARTESIAN_POINT('Origin',(0.,285.,0.));
#4932=CARTESIAN_POINT('Origin',(-37.,285.,4.));
#4933=CARTESIAN_POINT('',(-37.,275.,6.00000000000001));
#4934=CARTESIAN_POINT('',(-37.,345.,6.00000000000001));
#4935=CARTESIAN_POINT('',(-37.,275.,-5.99999999999999));
#4936=CARTESIAN_POINT('',(-37.,345.,-5.99999999999999));
#4937=CARTESIAN_POINT('',(-37.,275.,4.));
#4938=CARTESIAN_POINT('Origin',(0.,275.,0.));
#4939=CARTESIAN_POINT('',(-37.,275.,6.00000000000001));
#4940=CARTESIAN_POINT('',(-37.,275.,-5.99999999999999));
#4941=CARTESIAN_POINT('Origin',(0.,275.,0.));
#4942=CARTESIAN_POINT('',(37.,275.,-6.));
#4943=CARTESIAN_POINT('Origin',(0.,275.,0.));
#4944=CARTESIAN_POINT('Origin',(37.,345.,-6.));
#4945=CARTESIAN_POINT('',(-37.001,300.,-6.));
#4946=CARTESIAN_POINT('Origin',(-37.,345.,6.00000000000001));
#4947=CARTESIAN_POINT('Origin',(-37.,345.,-5.99999999999999));
#4948=CARTESIAN_POINT('Origin',(0.,0.,4.));
#4949=CARTESIAN_POINT('',(22.,335.,4.));
#4950=CARTESIAN_POINT('',(22.,329.539392014169,4.));
#4951=CARTESIAN_POINT('',(22.,335.,4.));
#4952=CARTESIAN_POINT('Origin',(32.,329.539392014169,4.));
#4953=CARTESIAN_POINT('',(-37.001,300.,4.));
#4954=CARTESIAN_POINT('',(63.8748866352591,335.,4.));
#4955=CARTESIAN_POINT('',(-37.,335.,4.));
#4956=CARTESIAN_POINT('',(143.521102017646,349.043776683232,4.));
#4957=CARTESIAN_POINT('',(64.7364817766693,335.151922469878,4.));
#4958=CARTESIAN_POINT('',(141.784620240977,358.891854213354,4.));
#4959=CARTESIAN_POINT('',(141.784620240977,358.891854213354,4.));
#4960=CARTESIAN_POINT('',(63.,345.,4.));
#4961=CARTESIAN_POINT('',(-37.,335.,4.));
#4962=CARTESIAN_POINT('Origin',(0.,0.,-4.));
#4963=CARTESIAN_POINT('',(22.,329.539392014169,-4.));
#4964=CARTESIAN_POINT('Origin',(32.,329.539392014169,-4.));
#4965=CARTESIAN_POINT('',(22.,335.,-4.));
#4966=CARTESIAN_POINT('',(22.,335.,-4.));
#4967=CARTESIAN_POINT('',(11.842719282327,335.,-4.));
#4968=CARTESIAN_POINT('',(-37.,335.,-4.));
#4969=CARTESIAN_POINT('',(11.842719282327,335.,-4.));
#4970=CARTESIAN_POINT('',(141.784620240977,358.891854213354,-4.));
#4971=CARTESIAN_POINT('',(63.,345.,-4.));
#4972=CARTESIAN_POINT('',(143.521102017646,349.043776683232,-4.));
#4973=CARTESIAN_POINT('',(141.784620240977,358.891854213354,-4.));
#4974=CARTESIAN_POINT('',(63.8748866352591,335.,-4.));
#4975=CARTESIAN_POINT('',(64.7364817766693,335.151922469878,-4.));
#4976=CARTESIAN_POINT('',(-37.,335.,-4.));
#4977=CARTESIAN_POINT('',(-37.001,300.,-4.));
#4978=CARTESIAN_POINT('Origin',(-37.,335.,4.));
#4979=CARTESIAN_POINT('',(22.,335.,-25.2132034355964));
#4980=CARTESIAN_POINT('Origin',(0.,335.,0.));
#4981=CARTESIAN_POINT('Origin',(-37.,335.,4.));
#4982=CARTESIAN_POINT('',(63.8748866352591,335.,4.));
#4983=CARTESIAN_POINT('Origin',(64.7364817766693,335.151922469878,4.));
#4984=CARTESIAN_POINT('',(143.521102017646,349.043776683232,4.));
#4985=CARTESIAN_POINT('Origin',(141.784620240977,358.891854213354,4.));
#4986=CARTESIAN_POINT('',(141.784620240977,358.891854213354,4.));
#4987=CARTESIAN_POINT('Origin',(63.,345.,4.));
#4988=CARTESIAN_POINT('Origin',(0.,335.,0.));
#4989=CARTESIAN_POINT('Origin',(-37.001,300.,-4.));
#4990=CARTESIAN_POINT('Origin',(-37.001,300.,4.));
#4991=CARTESIAN_POINT('Origin',(22.,335.,-25.2132034355964));
#4992=CARTESIAN_POINT('',(22.,329.539392014169,4.));
#4993=CARTESIAN_POINT('Origin',(32.,329.539392014169,-25.2132034355964));
#14065=UNCERTAINTY_MEASURE_WITH_UNIT(LENGTH_MEASURE(0.01),#14085,
'DISTANCE_ACCURACY_VALUE',
'Maximum model space distance between geometric entities at asserted c
onnectivities');
#14073=UNCERTAINTY_MEASURE_WITH_UNIT(LENGTH_MEASURE(0.01),#14085,
'DISTANCE_ACCURACY_VALUE',
'Maximum model space distance between geometric entities at asserted c
onnectivities');
#14076=(
GEOMETRIC_REPRESENTATION_CONTEXT(3)
GLOBAL_UNCERTAINTY_ASSIGNED_CONTEXT((#14065))
GLOBAL_UNIT_ASSIGNED_CONTEXT((#14085,#14087,#14088))
REPRESENTATION_CONTEXT('','3D')
);
#14084=(
GEOMETRIC_REPRESENTATION_CONTEXT(3)
GLOBAL_UNCERTAINTY_ASSIGNED_CONTEXT((#14073))
GLOBAL_UNIT_ASSIGNED_CONTEXT((#14085,#14087,#14088))
REPRESENTATION_CONTEXT('','3D')
);
#14085=(
LENGTH_UNIT()
NAMED_UNIT(*)
SI_UNIT(.MILLI.,.METRE.)
);
#14087=(
NAMED_UNIT(*)
PLANE_ANGLE_UNIT()
SI_UNIT($,.RADIAN.)
);
#14088=(
NAMED_UNIT(*)
SI_UNIT($,.STERADIAN.)
SOLID_ANGLE_UNIT()
);
#14091=SHAPE_DEFINITION_REPRESENTATION(#14101,#14121);
#14101=PRODUCT_DEFINITION_SHAPE('',$,#14132);
#14121=SHAPE_REPRESENTATION('',(#3597),#14076);
#14129=PRODUCT_DEFINITION_CONTEXT('part definition',#14161,'design');
#14132=PRODUCT_DEFINITION('head','head',#14142,#14129);
#14142=PRODUCT_DEFINITION_FORMATION('',$,#14165);
#14161=APPLICATION_CONTEXT(
'Core Data for Automotive Mechanical Design Process');
#14162=PRODUCT_CONTEXT('part definition',#14161,'mechanical');
#14165=PRODUCT('head','head',$,(#14162));
#14175=PRESENTATION_STYLE_ASSIGNMENT((#14181));
#14181=SURFACE_STYLE_USAGE(.BOTH.,#14187);
#14187=SURFACE_SIDE_STYLE('',(#14193));
#14193=SURFACE_STYLE_FILL_AREA(#14199);
#14199=FILL_AREA_STYLE('Opaque(227,224,212)',(#14205));
#14205=FILL_AREA_STYLE_COLOUR('Opaque(227,224,212)',#14211);
#14211=COLOUR_RGB('Opaque(227,224,212)',0.890196078431372,0.87843137254902,
0.831372549019608);
ENDSEC;
END-ISO-10303-21;
